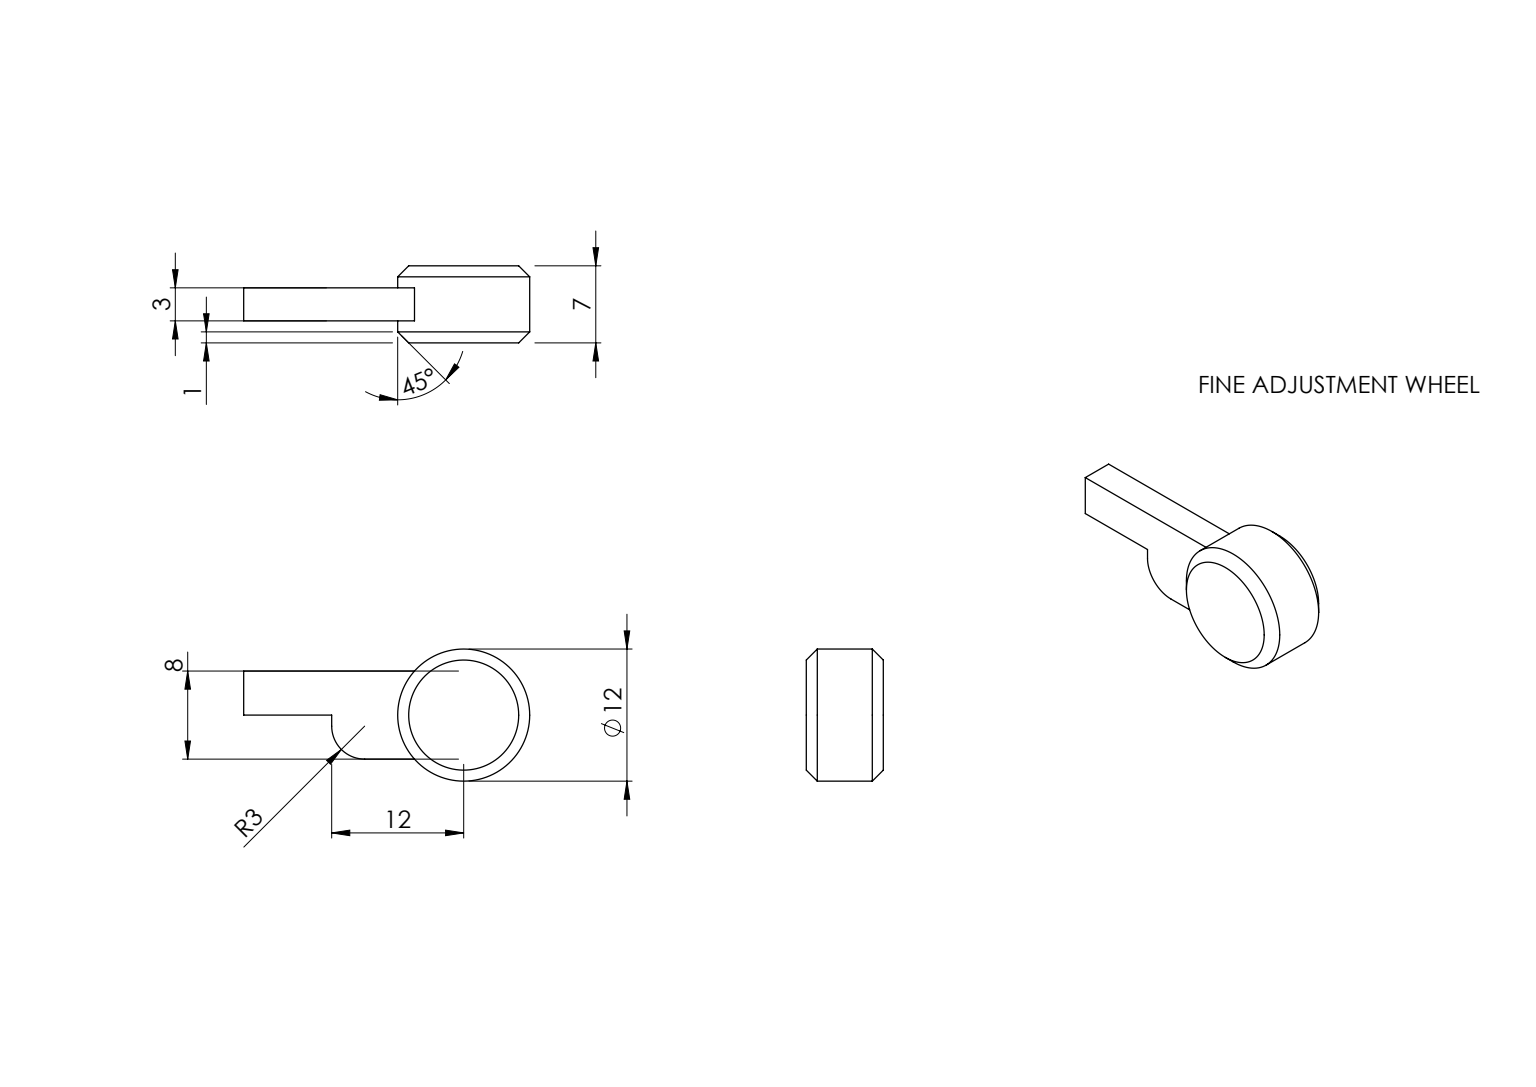
ISO-10303-21;
HEADER;
FILE_DESCRIPTION (('STEP AP214'),
    '1' );
FILE_NAME ('fine adjustment wheel.step',
    '2026-10-27T04:40:18',
    ( '' ),
    ( '' ),
    'SwSTEP 2.0',
    'SolidWorks 2026',
    '' );
FILE_SCHEMA (( 'AUTOMOTIVE_DESIGN' ));
ENDSEC;

DATA;
#10=ORIENTED_EDGE ( 'NONE', *, *, #8889, .F. ) ;
#13=ADVANCED_FACE ( 'NONE', ( #1458 ), #5708, .T. ) ;
#36=DIRECTION ( 'NONE',  ( 1.000000000000000000, 0.000000000000000000, 0.000000000000000000 ) ) ;
#47=DIRECTION ( 'NONE',  ( -0.000000000000000000, -0.000000000000000000, -1.000000000000000000 ) ) ;
#49=EDGE_LOOP ( 'NONE', ( #4259, #9067, #9089, #3500, #4349, #3630, #6139, #9782 ) ) ;
#70=CARTESIAN_POINT ( 'NONE',  ( -37.99999999999999289, -14.00000000000000888, -2.000000000000000000 ) ) ;
#86=ORIENTED_EDGE ( 'NONE', *, *, #4258, .T. ) ;
#91=EDGE_CURVE ( 'NONE', #7478, #353, #1465, .T. ) ;
#153=EDGE_CURVE ( 'NONE', #9355, #9315, #9914, .T. ) ;
#179=ADVANCED_BREP_SHAPE_REPRESENTATION ( '', ( #4912, #2307 ), #5679 ) ;
#216=ORIENTED_EDGE ( 'NONE', *, *, #8132, .T. ) ;
#224=VECTOR ( 'NONE', #3060, 999.9999999999998863 ) ;
#242=AXIS2_PLACEMENT_3D ( 'NONE', #968, #2330, #9109 ) ;
#274=LINE ( 'NONE', #989, #4138 ) ;
#291=CARTESIAN_POINT ( 'NONE',  ( -49.99999999999998579, -14.00000000000001243, 0.000000000000000000 ) ) ;
#300=ORIENTED_EDGE ( 'NONE', *, *, #8132, .F. ) ;
#327=AXIS2_PLACEMENT_3D ( 'NONE', #3024, #4508, #7911 ) ;
#339=EDGE_CURVE ( 'NONE', #1405, #2680, #6609, .T. ) ;
#353=VERTEX_POINT ( 'NONE', #8565 ) ;
#365=STYLED_ITEM ( 'NONE', ( #4697 ), #179 ) ;
#405=ORIENTED_EDGE ( 'NONE', *, *, #8852, .F. ) ;
#438=ORIENTED_EDGE ( 'NONE', *, *, #7786, .T. ) ;
#508=EDGE_CURVE ( 'NONE', #7478, #5442, #2848, .T. ) ;
#517=ORIENTED_EDGE ( 'NONE', *, *, #8212, .T. ) ;
#530=SHAPE_DEFINITION_REPRESENTATION ( #1480, #9271 ) ;
#531=DIRECTION ( 'NONE',  ( -1.000000000000000000, 0.000000000000000000, 0.000000000000000000 ) ) ;
#580=AXIS2_PLACEMENT_3D ( 'NONE', #1728, #9502, #4442 ) ;
#618=CARTESIAN_POINT ( 'NONE',  ( -37.99999999999999289, -14.00000000000000888, -0.9999999999999947820 ) ) ;
#626=CARTESIAN_POINT ( 'NONE',  ( -37.99999999999999289, -14.00000000000000888, -0.9999999999999947820 ) ) ;
#627=FACE_OUTER_BOUND ( 'NONE', #8133, .T. ) ;
#640=ADVANCED_FACE ( 'NONE', ( #10832 ), #2433, .T. ) ;
#668=CIRCLE ( 'NONE', #1009, 3.000000000000002665 ) ;
#712=EDGE_LOOP ( 'NONE', ( #5700, #5291 ) ) ;
#713=CARTESIAN_POINT ( 'NONE',  ( -57.99999999999998579, -10.00000000000000888, 0.000000000000000000 ) ) ;
#741=EDGE_CURVE ( 'NONE', #9355, #2941, #7719, .T. ) ;
#812=ORIENTED_EDGE ( 'NONE', *, *, #91, .F. ) ;
#866=CARTESIAN_POINT ( 'NONE',  ( -49.99999999999998579, -14.00000000000001243, 3.000000000000000000 ) ) ;
#903=DIRECTION ( 'NONE',  ( -1.000000000000000000, 0.000000000000000000, 0.000000000000000000 ) ) ;
#908=CARTESIAN_POINT ( 'NONE',  ( -43.00000000000000711, -14.00000000000000888, 5.000000000000000000 ) ) ;
#931=FACE_OUTER_BOUND ( 'NONE', #8908, .T. ) ;
#933=ORIENTED_EDGE ( 'NONE', *, *, #3473, .F. ) ;
#937=DIRECTION ( 'NONE',  ( -0.000000000000000000, -0.000000000000000000, -1.000000000000000000 ) ) ;
#968=CARTESIAN_POINT ( 'NONE',  ( -46.99999999999998579, -15.00000000000001066, 0.000000000000000000 ) ) ;
#989=CARTESIAN_POINT ( 'NONE',  ( -31.99999999999998579, -14.00000000000000888, -0.9999999999999947820 ) ) ;
#1001=APPLICATION_CONTEXT ( 'automotive_design' ) ;
#1009=AXIS2_PLACEMENT_3D ( 'NONE', #2485, #7596, #1705 ) ;
#1111=CARTESIAN_POINT ( 'NONE',  ( -46.99999999999998579, -18.00000000000001066, 0.000000000000000000 ) ) ;
#1122=CIRCLE ( 'NONE', #2538, 6.000000000000005329 ) ;
#1146=LINE ( 'NONE', #4527, #1576 ) ;
#1201=( NAMED_UNIT ( * ) SI_UNIT ( $, .STERADIAN. ) SOLID_ANGLE_UNIT ( ) );
#1208=DIRECTION ( 'NONE',  ( -0.000000000000000000, 0.000000000000000000, 1.000000000000000000 ) ) ;
#1210=DIRECTION ( 'NONE',  ( -0.000000000000000000, -0.000000000000000000, -1.000000000000000000 ) ) ;
#1256=MECHANICAL_DESIGN_GEOMETRIC_PRESENTATION_REPRESENTATION('',(#365),#3726);
#1265=SURFACE_SIDE_STYLE ('',( #8878 ) ) ;
#1327=SURFACE_STYLE_USAGE ( .BOTH. , #1265 ) ;
#1350=LINE ( 'NONE', #3214, #9205 ) ;
#1354=ORIENTED_EDGE ( 'NONE', *, *, #2995, .F. ) ;
#1391=CARTESIAN_POINT ( 'NONE',  ( -43.00000000000000711, -14.00000000000000888, 5.000000000000000000 ) ) ;
#1400=DIRECTION ( 'NONE',  ( 0.000000000000000000, 0.000000000000000000, 1.000000000000000000 ) ) ;
#1405=VERTEX_POINT ( 'NONE', #2148 ) ;
#1445=DIRECTION ( 'NONE',  ( 1.000000000000000000, 0.000000000000000000, 0.000000000000000000 ) ) ;
#1458=FACE_OUTER_BOUND ( 'NONE', #2511, .T. ) ;
#1462=( NAMED_UNIT ( * ) PLANE_ANGLE_UNIT ( ) SI_UNIT ( $, .RADIAN. ) );
#1465=CIRCLE ( 'NONE', #4462, 6.000000000000005329 ) ;
#1480=PRODUCT_DEFINITION_SHAPE ( 'NONE', 'NONE',  #3253 ) ;
#1506=DIRECTION ( 'NONE',  ( 0.000000000000000000, -1.000000000000000000, 0.000000000000000000 ) ) ;
#1550=EDGE_CURVE ( 'NONE', #3881, #2721, #10065, .T. ) ;
#1552=DIRECTION ( 'NONE',  ( 1.000000000000000000, 0.000000000000000000, -0.000000000000000000 ) ) ;
#1576=VECTOR ( 'NONE', #6088, 1000.000000000000000 ) ;
#1590=ORIENTED_EDGE ( 'NONE', *, *, #8473, .F. ) ;
#1597=LINE ( 'NONE', #10875, #4744 ) ;
#1613=DIRECTION ( 'NONE',  ( 0.000000000000000000, 0.000000000000000000, -1.000000000000000000 ) ) ;
#1629=CLOSED_SHELL ( 'NONE', ( #3641, #13, #7424, #7023, #3241, #9816, #9154, #8281, #8359, #2977, #2527, #640, #4769, #7997, #5715, #2128 ) ) ;
#1683=PLANE ( 'NONE',  #2131 ) ;
#1705=DIRECTION ( 'NONE',  ( 1.000000000000000000, 0.000000000000000000, 0.000000000000000000 ) ) ;
#1706=DIRECTION ( 'NONE',  ( 1.000000000000000000, 0.000000000000000000, 0.000000000000000000 ) ) ;
#1728=CARTESIAN_POINT ( 'NONE',  ( -37.99999999999999289, -14.00000000000000888, -2.000000000000000000 ) ) ;
#1738=DIRECTION ( 'NONE',  ( 0.000000000000000000, 0.000000000000000000, 1.000000000000000000 ) ) ;
#1745=FACE_OUTER_BOUND ( 'NONE', #9362, .T. ) ;
#1753=LINE ( 'NONE', #4344, #8240 ) ;
#1799=CARTESIAN_POINT ( 'NONE',  ( -46.99999999999998579, -15.00000000000001066, 3.000000000000000000 ) ) ;
#1808=CARTESIAN_POINT ( 'NONE',  ( -42.47213595499957961, -18.00000000000001066, 3.000000000000000000 ) ) ;
#1866=CARTESIAN_POINT ( 'NONE',  ( -49.99999999999998579, -18.00000000000001066, 3.000000000000000000 ) ) ;
#1873=APPLICATION_CONTEXT ( 'automotive_design' ) ;
#1881=FACE_OUTER_BOUND ( 'NONE', #4804, .T. ) ;
#1932=ORIENTED_EDGE ( 'NONE', *, *, #7786, .F. ) ;
#1992=DIRECTION ( 'NONE',  ( -0.000000000000000000, 0.000000000000000000, -1.000000000000000000 ) ) ;
#2011=LINE ( 'NONE', #3612, #5286 ) ;
#2028=AXIS2_PLACEMENT_3D ( 'NONE', #10381, #937, #2725 ) ;
#2094=DIRECTION ( 'NONE',  ( 0.000000000000000000, -0.000000000000000000, 1.000000000000000000 ) ) ;
#2101=CARTESIAN_POINT ( 'NONE',  ( 0.000000000000000000, 0.000000000000000000, 3.000000000000000000 ) ) ;
#2128=ADVANCED_FACE ( 'NONE', ( #1745 ), #2802, .T. ) ;
#2131=AXIS2_PLACEMENT_3D ( 'NONE', #7736, #5056, #2617 ) ;
#2148=CARTESIAN_POINT ( 'NONE',  ( -32.99999999999998579, -14.00000000000000888, -2.000000000000000000 ) ) ;
#2186=DIRECTION ( 'NONE',  ( 1.000000000000000000, -1.734723475976805517E-15, 0.000000000000000000 ) ) ;
#2199=FACE_OUTER_BOUND ( 'NONE', #4921, .T. ) ;
#2301=DIRECTION ( 'NONE',  ( 0.000000000000000000, 0.000000000000000000, -1.000000000000000000 ) ) ;
#2307=AXIS2_PLACEMENT_3D ( 'NONE', #5193, #3646, #1706 ) ;
#2314=CIRCLE ( 'NONE', #9227, 6.000000000000005329 ) ;
#2330=DIRECTION ( 'NONE',  ( 0.000000000000000000, -0.000000000000000000, -1.000000000000000000 ) ) ;
#2337=LINE ( 'NONE', #9118, #4782 ) ;
#2343=VECTOR ( 'NONE', #8296, 1000.000000000000000 ) ;
#2349=DIRECTION ( 'NONE',  ( 0.000000000000000000, 0.000000000000000000, -1.000000000000000000 ) ) ;
#2386=DIRECTION ( 'NONE',  ( -0.000000000000000000, -0.000000000000000000, 1.000000000000000000 ) ) ;
#2387=DIRECTION ( 'NONE',  ( -1.000000000000000000, 0.000000000000000000, 0.000000000000000000 ) ) ;
#2402=DIRECTION ( 'NONE',  ( 0.000000000000000000, 0.000000000000000000, 1.000000000000000000 ) ) ;
#2428=AXIS2_PLACEMENT_3D ( 'NONE', #6380, #8939, #3823 ) ;
#2433=PLANE ( 'NONE',  #7154 ) ;
#2436=EDGE_CURVE ( 'NONE', #4203, #4184, #3595, .T. ) ;
#2442=( LENGTH_UNIT ( ) NAMED_UNIT ( * ) SI_UNIT ( .MILLI., .METRE. ) );
#2454=CARTESIAN_POINT ( 'NONE',  ( -44.00000000000000000, -14.00000000000000888, -0.9999999999999947820 ) ) ;
#2457=EDGE_CURVE ( 'NONE', #5442, #2721, #1122, .T. ) ;
#2458=CONICAL_SURFACE ( 'NONE', #10080, 5.000000000000018652, 0.7853981633974430610 ) ;
#2485=CARTESIAN_POINT ( 'NONE',  ( -46.99999999999998579, -15.00000000000001066, 3.000000000000000000 ) ) ;
#2507=DIRECTION ( 'NONE',  ( -0.000000000000000000, -0.000000000000000000, -1.000000000000000000 ) ) ;
#2511=EDGE_LOOP ( 'NONE', ( #1590, #7595, #1354, #8774 ) ) ;
#2527=ADVANCED_FACE ( 'NONE', ( #9231 ), #2606, .T. ) ;
#2538=AXIS2_PLACEMENT_3D ( 'NONE', #5888, #3381, #8289 ) ;
#2606=CYLINDRICAL_SURFACE ( 'NONE', #2028, 6.000000000000005329 ) ;
#2617=DIRECTION ( 'NONE',  ( 0.000000000000000000, -0.000000000000000000, -1.000000000000000000 ) ) ;
#2647=EDGE_CURVE ( 'NONE', #1405, #9106, #274, .T. ) ;
#2657=ORIENTED_EDGE ( 'NONE', *, *, #6128, .F. ) ;
#2673=DIRECTION ( 'NONE',  ( 0.000000000000000000, -0.000000000000000000, 1.000000000000000000 ) ) ;
#2680=VERTEX_POINT ( 'NONE', #5150 ) ;
#2690=DIRECTION ( 'NONE',  ( -0.000000000000000000, 0.000000000000000000, -1.000000000000000000 ) ) ;
#2691=ORIENTED_EDGE ( 'NONE', *, *, #2647, .T. ) ;
#2712=ORIENTED_EDGE ( 'NONE', *, *, #339, .F. ) ;
#2721=VERTEX_POINT ( 'NONE', #9785 ) ;
#2722=AXIS2_PLACEMENT_3D ( 'NONE', #618, #6864, #3357 ) ;
#2725=DIRECTION ( 'NONE',  ( -1.000000000000000000, 0.000000000000000000, 0.000000000000000000 ) ) ;
#2734=VERTEX_POINT ( 'NONE', #6508 ) ;
#2768=CARTESIAN_POINT ( 'NONE',  ( -57.99999999999998579, -10.00000000000000888, 3.000000000000000000 ) ) ;
#2793=EDGE_CURVE ( 'NONE', #4184, #353, #7173, .T. ) ;
#2795=ORIENTED_EDGE ( 'NONE', *, *, #8073, .T. ) ;
#2802=CYLINDRICAL_SURFACE ( 'NONE', #5740, 3.000000000000002665 ) ;
#2819=CARTESIAN_POINT ( 'NONE',  ( -57.99999999999998579, -10.00000000000000888, 0.000000000000000000 ) ) ;
#2834=ORIENTED_EDGE ( 'NONE', *, *, #7357, .T. ) ;
#2848=LINE ( 'NONE', #10615, #9097 ) ;
#2850=DIRECTION ( 'NONE',  ( 0.000000000000000000, -0.000000000000000000, -1.000000000000000000 ) ) ;
#2880=CARTESIAN_POINT ( 'NONE',  ( -49.99999999999998579, -14.00000000000001243, 3.000000000000000000 ) ) ;
#2902=EDGE_CURVE ( 'NONE', #3086, #4883, #1753, .T. ) ;
#2916=LINE ( 'NONE', #6304, #5810 ) ;
#2941=VERTEX_POINT ( 'NONE', #1808 ) ;
#2959=DIRECTION ( 'NONE',  ( 0.000000000000000000, -1.000000000000000000, 0.000000000000000000 ) ) ;
#2977=ADVANCED_FACE ( 'NONE', ( #6925 ), #3524, .F. ) ;
#2995=EDGE_CURVE ( 'NONE', #9106, #8034, #6093, .T. ) ;
#3004=MECHANICAL_DESIGN_GEOMETRIC_PRESENTATION_REPRESENTATION('',(#6552),#5273);
#3024=CARTESIAN_POINT ( 'NONE',  ( -37.99999999999999289, -14.00000000000000888, -0.9999999999999947820 ) ) ;
#3034=ORIENTED_EDGE ( 'NONE', *, *, #2793, .F. ) ;
#3060=DIRECTION ( 'NONE',  ( -0.7071067811865439090, 0.000000000000000000, -0.7071067811865512365 ) ) ;
#3069=ORIENTED_EDGE ( 'NONE', *, *, #8889, .T. ) ;
#3077=ORIENTED_EDGE ( 'NONE', *, *, #2902, .T. ) ;
#3078=CARTESIAN_POINT ( 'NONE',  ( -31.99999999999997868, -14.00000000000000888, -0.9999999999999947820 ) ) ;
#3086=VERTEX_POINT ( 'NONE', #5179 ) ;
#3094=EDGE_CURVE ( 'NONE', #9315, #7434, #8946, .T. ) ;
#3096=( NAMED_UNIT ( * ) PLANE_ANGLE_UNIT ( ) SI_UNIT ( $, .RADIAN. ) );
#3135=DIRECTION ( 'NONE',  ( 1.000000000000000000, 0.000000000000000000, 0.000000000000000000 ) ) ;
#3175=DIRECTION ( 'NONE',  ( 1.000000000000000000, 0.000000000000000000, 0.000000000000000000 ) ) ;
#3214=CARTESIAN_POINT ( 'NONE',  ( -57.99999999999998579, -10.00000000000000888, 3.000000000000000000 ) ) ;
#3241=ADVANCED_FACE ( 'NONE', ( #9702 ), #6981, .F. ) ;
#3253=PRODUCT_DEFINITION ( 'UNKNOWN', '', #7291, #4620 ) ;
#3271=UNCERTAINTY_MEASURE_WITH_UNIT (LENGTH_MEASURE( 1.000000000000000082E-05 ), #2442, 'distance_accuracy_value', 'NONE');
#3305=EDGE_CURVE ( 'NONE', #5709, #3086, #6491, .T. ) ;
#3337=ORIENTED_EDGE ( 'NONE', *, *, #3473, .T. ) ;
#3357=DIRECTION ( 'NONE',  ( 1.000000000000000000, 0.000000000000000000, 0.000000000000000000 ) ) ;
#3381=DIRECTION ( 'NONE',  ( 0.000000000000000000, -0.000000000000000000, -1.000000000000000000 ) ) ;
#3386=LINE ( 'NONE', #3496, #3889 ) ;
#3430=DIRECTION ( 'NONE',  ( 1.000000000000000000, 0.000000000000000000, 0.000000000000000000 ) ) ;
#3439=CARTESIAN_POINT ( 'NONE',  ( -57.99999999999998579, -14.00000000000001243, 3.000000000000000000 ) ) ;
#3473=EDGE_CURVE ( 'NONE', #2734, #7921, #9567, .T. ) ;
#3496=CARTESIAN_POINT ( 'NONE',  ( -44.00000000000000000, -14.00000000000000888, 5.000000000000000000 ) ) ;
#3497=VECTOR ( 'NONE', #7882, 1000.000000000000000 ) ;
#3500=ORIENTED_EDGE ( 'NONE', *, *, #8212, .F. ) ;
#3524=PLANE ( 'NONE',  #8061 ) ;
#3534=COLOUR_RGB ( '',0.8941176470588234615, 0.8941176470588234615, 0.8941176470588234615 ) ;
#3583=AXIS2_PLACEMENT_3D ( 'NONE', #1866, #4468, #2094 ) ;
#3595=CIRCLE ( 'NONE', #5912, 5.000000000000018652 ) ;
#3612=CARTESIAN_POINT ( 'NONE',  ( -49.99999999999998579, -10.00000000000000888, 0.000000000000000000 ) ) ;
#3630=ORIENTED_EDGE ( 'NONE', *, *, #7165, .T. ) ;
#3641=ADVANCED_FACE ( 'NONE', ( #627 ), #8743, .T. ) ;
#3646=DIRECTION ( 'NONE',  ( 0.000000000000000000, 0.000000000000000000, 1.000000000000000000 ) ) ;
#3689=CARTESIAN_POINT ( 'NONE',  ( -32.99999999999997158, -14.00000000000000888, 5.000000000000000000 ) ) ;
#3726=( GEOMETRIC_REPRESENTATION_CONTEXT ( 3 ) GLOBAL_UNCERTAINTY_ASSIGNED_CONTEXT ( ( #7376 ) ) GLOBAL_UNIT_ASSIGNED_CONTEXT ( ( #8986, #3096, #4859 ) ) REPRESENTATION_CONTEXT ( 'NONE', 'WORKASPACE' ) );
#3774=VECTOR ( 'NONE', #3430, 1000.000000000000000 ) ;
#3809=EDGE_LOOP ( 'NONE', ( #3826, #2795, #9159, #7912 ) ) ;
#3822=VERTEX_POINT ( 'NONE', #7558 ) ;
#3823=DIRECTION ( 'NONE',  ( 1.000000000000000000, 0.000000000000000000, 0.000000000000000000 ) ) ;
#3826=ORIENTED_EDGE ( 'NONE', *, *, #6064, .T. ) ;
#3868=CIRCLE ( 'NONE', #9899, 5.000000000000018652 ) ;
#3878=DIRECTION ( 'NONE',  ( 0.000000000000000000, 0.000000000000000000, 1.000000000000000000 ) ) ;
#3881=VERTEX_POINT ( 'NONE', #5991 ) ;
#3889=VECTOR ( 'NONE', #2507, 1000.000000000000000 ) ;
#3906=AXIS2_PLACEMENT_3D ( 'NONE', #6884, #47, #10933 ) ;
#3915=CONICAL_SURFACE ( 'NONE', #5308, 6.000000000000005329, 0.7853981633974479459 ) ;
#3938=DIRECTION ( 'NONE',  ( 0.000000000000000000, -1.000000000000000000, 0.000000000000000000 ) ) ;
#3949=AXIS2_PLACEMENT_3D ( 'NONE', #10889, #1613, #2387 ) ;
#4033=CIRCLE ( 'NONE', #4565, 5.000000000000004441 ) ;
#4087=EDGE_CURVE ( 'NONE', #4203, #7478, #9887, .T. ) ;
#4127=VECTOR ( 'NONE', #10514, 1000.000000000000000 ) ;
#4138=VECTOR ( 'NONE', #7055, 1000.000000000000000 ) ;
#4147=ORIENTED_EDGE ( 'NONE', *, *, #8394, .F. ) ;
#4156=ORIENTED_EDGE ( 'NONE', *, *, #2436, .T. ) ;
#4169=DIRECTION ( 'NONE',  ( -0.7071067811865472397, 8.659560562354929160E-17, 0.7071067811865479058 ) ) ;
#4184=VERTEX_POINT ( 'NONE', #3689 ) ;
#4186=DIRECTION ( 'NONE',  ( 1.000000000000000000, 0.000000000000000000, -0.000000000000000000 ) ) ;
#4203=VERTEX_POINT ( 'NONE', #908 ) ;
#4209=CARTESIAN_POINT ( 'NONE',  ( -37.99999999999999289, -14.00000000000000888, 5.000000000000000000 ) ) ;
#4258=EDGE_CURVE ( 'NONE', #5709, #8064, #6196, .T. ) ;
#4259=ORIENTED_EDGE ( 'NONE', *, *, #10324, .F. ) ;
#4302=DIRECTION ( 'NONE',  ( -0.000000000000000000, -0.000000000000000000, 1.000000000000000000 ) ) ;
#4344=CARTESIAN_POINT ( 'NONE',  ( -57.99999999999998579, -14.00000000000001243, 0.000000000000000000 ) ) ;
#4349=ORIENTED_EDGE ( 'NONE', *, *, #9274, .T. ) ;
#4351=CARTESIAN_POINT ( 'NONE',  ( -49.99999999999998579, -15.00000000000001066, 3.000000000000000000 ) ) ;
#4442=DIRECTION ( 'NONE',  ( 1.000000000000000000, 0.000000000000000000, 0.000000000000000000 ) ) ;
#4444=DIRECTION ( 'NONE',  ( 0.000000000000000000, -0.000000000000000000, -1.000000000000000000 ) ) ;
#4462=AXIS2_PLACEMENT_3D ( 'NONE', #8254, #2349, #3135 ) ;
#4468=DIRECTION ( 'NONE',  ( 0.000000000000000000, 1.000000000000000000, 0.000000000000000000 ) ) ;
#4488=EDGE_LOOP ( 'NONE', ( #4156, #7221 ) ) ;
#4505=CARTESIAN_POINT ( 'NONE',  ( -57.99999999999998579, -10.00000000000000888, 3.000000000000000000 ) ) ;
#4508=DIRECTION ( 'NONE',  ( -0.000000000000000000, -0.000000000000000000, 1.000000000000000000 ) ) ;
#4527=CARTESIAN_POINT ( 'NONE',  ( -31.99999999999998579, -14.00000000000000888, 5.000000000000000000 ) ) ;
#4556=EDGE_LOOP ( 'NONE', ( #3077, #9544, #5564, #9901 ) ) ;
#4563=DIRECTION ( 'NONE',  ( 0.000000000000000000, 0.000000000000000000, -1.000000000000000000 ) ) ;
#4565=AXIS2_PLACEMENT_3D ( 'NONE', #8826, #1210, #4591 ) ;
#4588=DIRECTION ( 'NONE',  ( 1.000000000000000000, 0.000000000000000000, 0.000000000000000000 ) ) ;
#4591=DIRECTION ( 'NONE',  ( 1.000000000000000000, 0.000000000000000000, 0.000000000000000000 ) ) ;
#4617=DIRECTION ( 'NONE',  ( -0.000000000000000000, -0.000000000000000000, -1.000000000000000000 ) ) ;
#4620=PRODUCT_DEFINITION_CONTEXT ( 'detailed design', #1873, 'design' ) ;
#4697=PRESENTATION_STYLE_ASSIGNMENT (( #1327 ) ) ;
#4729=ORIENTED_EDGE ( 'NONE', *, *, #1550, .T. ) ;
#4744=VECTOR ( 'NONE', #10038, 1000.000000000000000 ) ;
#4748=CARTESIAN_POINT ( 'NONE',  ( -57.99999999999998579, -14.00000000000001243, 3.000000000000000000 ) ) ;
#4749=FILL_AREA_STYLE_COLOUR ( '', #3534 ) ;
#4769=ADVANCED_FACE ( 'NONE', ( #6123 ), #9345, .F. ) ;
#4782=VECTOR ( 'NONE', #1506, 1000.000000000000000 ) ;
#4804=EDGE_LOOP ( 'NONE', ( #438, #8620, #6062, #3337 ) ) ;
#4808=PLANE ( 'NONE',  #2428 ) ;
#4859=( NAMED_UNIT ( * ) SI_UNIT ( $, .STERADIAN. ) SOLID_ANGLE_UNIT ( ) );
#4883=VERTEX_POINT ( 'NONE', #291 ) ;
#4887=( NAMED_UNIT ( * ) SI_UNIT ( $, .STERADIAN. ) SOLID_ANGLE_UNIT ( ) );
#4892=EDGE_CURVE ( 'NONE', #8034, #9106, #8658, .T. ) ;
#4912=MANIFOLD_SOLID_BREP ( 'Fillet1', #1629 ) ;
#4921=EDGE_LOOP ( 'NONE', ( #3034, #7353, #9276, #405 ) ) ;
#4980=AXIS2_PLACEMENT_3D ( 'NONE', #70, #1738, #5112 ) ;
#4994=DIRECTION ( 'NONE',  ( 0.000000000000000000, 1.000000000000000000, 0.000000000000000000 ) ) ;
#5056=DIRECTION ( 'NONE',  ( 0.000000000000000000, -1.000000000000000000, 0.000000000000000000 ) ) ;
#5112=DIRECTION ( 'NONE',  ( 1.000000000000000000, 0.000000000000000000, -0.000000000000000000 ) ) ;
#5150=CARTESIAN_POINT ( 'NONE',  ( -43.00000000000000000, -14.00000000000000888, -2.000000000000000000 ) ) ;
#5176=CARTESIAN_POINT ( 'NONE',  ( -57.99999999999998579, -14.00000000000001243, 3.000000000000000000 ) ) ;
#5177=ORIENTED_EDGE ( 'NONE', *, *, #10324, .T. ) ;
#5178=VECTOR ( 'NONE', #2402, 1000.000000000000000 ) ;
#5179=CARTESIAN_POINT ( 'NONE',  ( -57.99999999999998579, -14.00000000000001243, 0.000000000000000000 ) ) ;
#5190=LINE ( 'NONE', #4351, #6219 ) ;
#5193=CARTESIAN_POINT ( 'NONE',  ( 0.000000000000000000, 0.000000000000000000, 0.000000000000000000 ) ) ;
#5201=ORIENTED_EDGE ( 'NONE', *, *, #7114, .T. ) ;
#5244=PLANE ( 'NONE',  #8470 ) ;
#5273=( GEOMETRIC_REPRESENTATION_CONTEXT ( 3 ) GLOBAL_UNCERTAINTY_ASSIGNED_CONTEXT ( ( #3271 ) ) GLOBAL_UNIT_ASSIGNED_CONTEXT ( ( #2442, #1462, #4887 ) ) REPRESENTATION_CONTEXT ( 'NONE', 'WORKASPACE' ) );
#5284=ORIENTED_EDGE ( 'NONE', *, *, #2793, .T. ) ;
#5286=VECTOR ( 'NONE', #2959, 1000.000000000000000 ) ;
#5291=ORIENTED_EDGE ( 'NONE', *, *, #8473, .T. ) ;
#5308=AXIS2_PLACEMENT_3D ( 'NONE', #5814, #4302, #36 ) ;
#5374=VECTOR ( 'NONE', #9002, 999.9999999999998863 ) ;
#5442=VERTEX_POINT ( 'NONE', #10043 ) ;
#5545=ORIENTED_EDGE ( 'NONE', *, *, #4892, .F. ) ;
#5564=ORIENTED_EDGE ( 'NONE', *, *, #4258, .F. ) ;
#5573=ORIENTED_EDGE ( 'NONE', *, *, #741, .T. ) ;
#5577=CARTESIAN_POINT ( 'NONE',  ( -37.99999999999999289, -14.00000000000000888, 5.000000000000000000 ) ) ;
#5642=DIRECTION ( 'NONE',  ( -0.000000000000000000, -0.000000000000000000, -1.000000000000000000 ) ) ;
#5658=ORIENTED_EDGE ( 'NONE', *, *, #8113, .T. ) ;
#5666=DIRECTION ( 'NONE',  ( -1.000000000000000000, -0.000000000000000000, -0.000000000000000000 ) ) ;
#5673=CIRCLE ( 'NONE', #8339, 6.000000000000005329 ) ;
#5679=( GEOMETRIC_REPRESENTATION_CONTEXT ( 3 ) GLOBAL_UNCERTAINTY_ASSIGNED_CONTEXT ( ( #6600 ) ) GLOBAL_UNIT_ASSIGNED_CONTEXT ( ( #10706, #10646, #1201 ) ) REPRESENTATION_CONTEXT ( 'NONE', 'WORKASPACE' ) );
#5689=LINE ( 'NONE', #2454, #9044 ) ;
#5694=EDGE_LOOP ( 'NONE', ( #10, #9413, #7170, #5973, #1932, #8095, #6662, #7528 ) ) ;
#5700=ORIENTED_EDGE ( 'NONE', *, *, #339, .T. ) ;
#5708=CONICAL_SURFACE ( 'NONE', #6255, 6.000000000000005329, 0.7853981633974479459 ) ;
#5709=VERTEX_POINT ( 'NONE', #7305 ) ;
#5715=ADVANCED_FACE ( 'NONE', ( #2199 ), #2458, .T. ) ;
#5740=AXIS2_PLACEMENT_3D ( 'NONE', #1799, #2690, #903 ) ;
#5761=ORIENTED_EDGE ( 'NONE', *, *, #2457, .F. ) ;
#5810=VECTOR ( 'NONE', #9686, 1000.000000000000000 ) ;
#5814=CARTESIAN_POINT ( 'NONE',  ( -37.99999999999999289, -14.00000000000000888, -0.9999999999999947820 ) ) ;
#5846=CARTESIAN_POINT ( 'NONE',  ( -42.47213595499957961, -10.00000000000000888, 5.000000000000000000 ) ) ;
#5870=CARTESIAN_POINT ( 'NONE',  ( -44.00000000000000711, -14.00000000000000888, -0.9999999999999947820 ) ) ;
#5884=ORIENTED_EDGE ( 'NONE', *, *, #153, .F. ) ;
#5886=EDGE_CURVE ( 'NONE', #6102, #8034, #3386, .T. ) ;
#5888=CARTESIAN_POINT ( 'NONE',  ( -37.99999999999999289, -14.00000000000000888, 3.000000000000000000 ) ) ;
#5901=FACE_OUTER_BOUND ( 'NONE', #6795, .T. ) ;
#5912=AXIS2_PLACEMENT_3D ( 'NONE', #4209, #10158, #3175 ) ;
#5937=CARTESIAN_POINT ( 'NONE',  ( -49.99999999999998579, -15.00000000000001066, 0.000000000000000000 ) ) ;
#5973=ORIENTED_EDGE ( 'NONE', *, *, #2902, .F. ) ;
#5987=AXIS2_PLACEMENT_3D ( 'NONE', #8089, #4563, #8917 ) ;
#5991=CARTESIAN_POINT ( 'NONE',  ( -42.47213595499957961, -10.00000000000000888, 0.000000000000000000 ) ) ;
#6062=ORIENTED_EDGE ( 'NONE', *, *, #7357, .F. ) ;
#6064=EDGE_CURVE ( 'NONE', #4883, #7434, #2011, .T. ) ;
#6088=DIRECTION ( 'NONE',  ( -0.000000000000000000, -0.000000000000000000, -1.000000000000000000 ) ) ;
#6093=CIRCLE ( 'NONE', #2722, 6.000000000000005329 ) ;
#6102=VERTEX_POINT ( 'NONE', #9005 ) ;
#6123=FACE_OUTER_BOUND ( 'NONE', #712, .T. ) ;
#6128=EDGE_CURVE ( 'NONE', #2721, #2734, #1350, .T. ) ;
#6139=ORIENTED_EDGE ( 'NONE', *, *, #5886, .T. ) ;
#6196=LINE ( 'NONE', #5176, #8387 ) ;
#6219=VECTOR ( 'NONE', #9210, 1000.000000000000000 ) ;
#6255=AXIS2_PLACEMENT_3D ( 'NONE', #626, #2386, #10781 ) ;
#6268=DIRECTION ( 'NONE',  ( -1.000000000000000000, -0.000000000000000000, -0.000000000000000000 ) ) ;
#6273=DIRECTION ( 'NONE',  ( 1.000000000000000000, 0.000000000000000000, -0.000000000000000000 ) ) ;
#6304=CARTESIAN_POINT ( 'NONE',  ( -49.99999999999998579, -18.00000000000001066, 0.000000000000000000 ) ) ;
#6380=CARTESIAN_POINT ( 'NONE',  ( 0.000000000000000000, 0.000000000000000000, 0.000000000000000000 ) ) ;
#6452=VERTEX_POINT ( 'NONE', #7542 ) ;
#6491=LINE ( 'NONE', #4748, #8380 ) ;
#6508=CARTESIAN_POINT ( 'NONE',  ( -57.99999999999998579, -10.00000000000000888, 3.000000000000000000 ) ) ;
#6514=CARTESIAN_POINT ( 'NONE',  ( -37.99999999999999289, -14.00000000000000888, 5.000000000000000000 ) ) ;
#6549=EDGE_CURVE ( 'NONE', #3881, #7921, #9593, .T. ) ;
#6552=STYLED_ITEM('',(#11006),#4912);
#6562=ORIENTED_EDGE ( 'NONE', *, *, #1550, .F. ) ;
#6599=SHAPE_REPRESENTATION_RELATIONSHIP ( 'NONE' , 'NONE' ,  #9271, #179 ) ;
#6600=UNCERTAINTY_MEASURE_WITH_UNIT (LENGTH_MEASURE( 1.000000000000000082E-05 ), #10706, 'distance_accuracy_value', 'NONE');
#6609=CIRCLE ( 'NONE', #580, 5.000000000000004441 ) ;
#6662=ORIENTED_EDGE ( 'NONE', *, *, #7114, .F. ) ;
#6688=EDGE_CURVE ( 'NONE', #2680, #8034, #5689, .T. ) ;
#6716=AXIS2_PLACEMENT_3D ( 'NONE', #2768, #6273, #1992 ) ;
#6795=EDGE_LOOP ( 'NONE', ( #6562, #7112, #933, #2657 ) ) ;
#6815=EDGE_LOOP ( 'NONE', ( #5658, #216, #5573, #517, #8607, #10223, #2834, #86 ) ) ;
#6864=DIRECTION ( 'NONE',  ( -0.000000000000000000, -0.000000000000000000, 1.000000000000000000 ) ) ;
#6884=CARTESIAN_POINT ( 'NONE',  ( -37.99999999999999289, -14.00000000000000888, 5.000000000000000000 ) ) ;
#6925=FACE_OUTER_BOUND ( 'NONE', #3809, .T. ) ;
#6981=PLANE ( 'NONE',  #3583 ) ;
#7023=ADVANCED_FACE ( 'NONE', ( #5901 ), #1683, .F. ) ;
#7040=DIRECTION ( 'NONE',  ( 0.000000000000000000, -0.000000000000000000, -1.000000000000000000 ) ) ;
#7055=DIRECTION ( 'NONE',  ( 0.7071067811865472397, 0.000000000000000000, 0.7071067811865479058 ) ) ;
#7057=CARTESIAN_POINT ( 'NONE',  ( -42.47213595499957961, -18.00000000000001066, 5.000000000000000000 ) ) ;
#7102=LINE ( 'NONE', #2880, #3497 ) ;
#7108=PLANE ( 'NONE',  #6716 ) ;
#7112=ORIENTED_EDGE ( 'NONE', *, *, #6549, .T. ) ;
#7114=EDGE_CURVE ( 'NONE', #6102, #3881, #5673, .T. ) ;
#7154=AXIS2_PLACEMENT_3D ( 'NONE', #6514, #1400, #1552 ) ;
#7165=EDGE_CURVE ( 'NONE', #6452, #6102, #2314, .T. ) ;
#7170=ORIENTED_EDGE ( 'NONE', *, *, #6064, .F. ) ;
#7173=LINE ( 'NONE', #10668, #5374 ) ;
#7175=LINE ( 'NONE', #7057, #7768 ) ;
#7221=ORIENTED_EDGE ( 'NONE', *, *, #8394, .T. ) ;
#7269=DIRECTION ( 'NONE',  ( 1.000000000000000000, 0.000000000000000000, 0.000000000000000000 ) ) ;
#7291=PRODUCT_DEFINITION_FORMATION_WITH_SPECIFIED_SOURCE ( 'ANY', '', #7422, .NOT_KNOWN. ) ;
#7297=ORIENTED_EDGE ( 'NONE', *, *, #5886, .F. ) ;
#7305=CARTESIAN_POINT ( 'NONE',  ( -57.99999999999998579, -14.00000000000001243, 3.000000000000000000 ) ) ;
#7353=ORIENTED_EDGE ( 'NONE', *, *, #2436, .F. ) ;
#7357=EDGE_CURVE ( 'NONE', #2734, #5709, #2337, .T. ) ;
#7376=UNCERTAINTY_MEASURE_WITH_UNIT (LENGTH_MEASURE( 1.000000000000000082E-05 ), #8986, 'distance_accuracy_value', 'NONE');
#7378=FACE_OUTER_BOUND ( 'NONE', #5694, .T. ) ;
#7386=LINE ( 'NONE', #8998, #8168 ) ;
#7422=PRODUCT ( 'fine adjustment wheel', 'fine adjustment wheel', '', ( #8973 ) ) ;
#7424=ADVANCED_FACE ( 'NONE', ( #931 ), #9378, .T. ) ;
#7434=VERTEX_POINT ( 'NONE', #5937 ) ;
#7470=ORIENTED_EDGE ( 'NONE', *, *, #6688, .F. ) ;
#7478=VERTEX_POINT ( 'NONE', #8439 ) ;
#7506=ORIENTED_EDGE ( 'NONE', *, *, #741, .F. ) ;
#7528=ORIENTED_EDGE ( 'NONE', *, *, #7165, .F. ) ;
#7542=CARTESIAN_POINT ( 'NONE',  ( -42.47213595499957961, -18.00000000000001066, 0.000000000000000000 ) ) ;
#7543=ORIENTED_EDGE ( 'NONE', *, *, #9274, .F. ) ;
#7558=CARTESIAN_POINT ( 'NONE',  ( -49.99999999999998579, -15.00000000000001066, 3.000000000000000000 ) ) ;
#7585=AXIS2_PLACEMENT_3D ( 'NONE', #7821, #7040, #7936 ) ;
#7588=DIRECTION ( 'NONE',  ( -0.000000000000000000, 0.000000000000000000, -1.000000000000000000 ) ) ;
#7595=ORIENTED_EDGE ( 'NONE', *, *, #6688, .T. ) ;
#7596=DIRECTION ( 'NONE',  ( -0.000000000000000000, 0.000000000000000000, 1.000000000000000000 ) ) ;
#7719=LINE ( 'NONE', #10255, #3774 ) ;
#7736=CARTESIAN_POINT ( 'NONE',  ( -57.99999999999998579, -10.00000000000000888, 3.000000000000000000 ) ) ;
#7754=DIRECTION ( 'NONE',  ( 1.000000000000000000, 0.000000000000000000, 0.000000000000000000 ) ) ;
#7768=VECTOR ( 'NONE', #9554, 1000.000000000000000 ) ;
#7786=EDGE_CURVE ( 'NONE', #7921, #3086, #7386, .T. ) ;
#7821=CARTESIAN_POINT ( 'NONE',  ( -37.99999999999999289, -14.00000000000000888, 3.000000000000000000 ) ) ;
#7828=ORIENTED_EDGE ( 'NONE', *, *, #4087, .F. ) ;
#7837=CARTESIAN_POINT ( 'NONE',  ( -46.99999999999998579, -18.00000000000001066, 3.000000000000000000 ) ) ;
#7882=DIRECTION ( 'NONE',  ( -0.000000000000000000, -0.000000000000000000, -1.000000000000000000 ) ) ;
#7905=DIRECTION ( 'NONE',  ( 1.000000000000000000, 0.000000000000000000, 0.000000000000000000 ) ) ;
#7911=DIRECTION ( 'NONE',  ( 1.000000000000000000, 0.000000000000000000, 0.000000000000000000 ) ) ;
#7912=ORIENTED_EDGE ( 'NONE', *, *, #8187, .T. ) ;
#7921=VERTEX_POINT ( 'NONE', #713 ) ;
#7936=DIRECTION ( 'NONE',  ( 1.000000000000000000, 0.000000000000000000, 0.000000000000000000 ) ) ;
#7964=ORIENTED_EDGE ( 'NONE', *, *, #91, .T. ) ;
#7997=ADVANCED_FACE ( 'NONE', ( #8482 ), #3915, .T. ) ;
#8034=VERTEX_POINT ( 'NONE', #5870 ) ;
#8061=AXIS2_PLACEMENT_3D ( 'NONE', #10132, #4186, #7588 ) ;
#8064=VERTEX_POINT ( 'NONE', #866 ) ;
#8073=EDGE_CURVE ( 'NONE', #7434, #3822, #5190, .T. ) ;
#8089=CARTESIAN_POINT ( 'NONE',  ( -37.99999999999999289, -14.00000000000000888, 3.999999999999999112 ) ) ;
#8095=ORIENTED_EDGE ( 'NONE', *, *, #6549, .F. ) ;
#8108=CARTESIAN_POINT ( 'NONE',  ( -37.99999999999999289, -14.00000000000000888, 5.000000000000000000 ) ) ;
#8113=EDGE_CURVE ( 'NONE', #8064, #3822, #1597, .T. ) ;
#8132=EDGE_CURVE ( 'NONE', #3822, #9355, #668, .T. ) ;
#8133=EDGE_LOOP ( 'NONE', ( #4147, #5284, #812, #7828 ) ) ;
#8168=VECTOR ( 'NONE', #3938, 1000.000000000000000 ) ;
#8187=EDGE_CURVE ( 'NONE', #8064, #4883, #7102, .T. ) ;
#8212=EDGE_CURVE ( 'NONE', #2941, #5442, #10060, .T. ) ;
#8240=VECTOR ( 'NONE', #1445, 1000.000000000000000 ) ;
#8254=CARTESIAN_POINT ( 'NONE',  ( -37.99999999999999289, -14.00000000000000888, 3.999999999999999112 ) ) ;
#8281=ADVANCED_FACE ( 'NONE', ( #10419 ), #5244, .T. ) ;
#8289=DIRECTION ( 'NONE',  ( 1.000000000000000000, -1.734723475976805517E-15, 0.000000000000000000 ) ) ;
#8296=DIRECTION ( 'NONE',  ( -0.000000000000000000, 0.000000000000000000, -1.000000000000000000 ) ) ;
#8339=AXIS2_PLACEMENT_3D ( 'NONE', #9794, #2850, #2186 ) ;
#8359=ADVANCED_FACE ( 'NONE', ( #7378 ), #4808, .F. ) ;
#8380=VECTOR ( 'NONE', #5642, 1000.000000000000000 ) ;
#8387=VECTOR ( 'NONE', #7754, 1000.000000000000000 ) ;
#8394=EDGE_CURVE ( 'NONE', #4184, #4203, #3868, .T. ) ;
#8398=FACE_OUTER_BOUND ( 'NONE', #4556, .T. ) ;
#8439=CARTESIAN_POINT ( 'NONE',  ( -44.00000000000000711, -14.00000000000000888, 3.999999999999999112 ) ) ;
#8470=AXIS2_PLACEMENT_3D ( 'NONE', #2101, #1208, #4588 ) ;
#8473=EDGE_CURVE ( 'NONE', #2680, #1405, #4033, .T. ) ;
#8482=FACE_OUTER_BOUND ( 'NONE', #9603, .T. ) ;
#8484=ORIENTED_EDGE ( 'NONE', *, *, #3094, .F. ) ;
#8565=CARTESIAN_POINT ( 'NONE',  ( -31.99999999999997868, -14.00000000000000888, 3.999999999999999112 ) ) ;
#8607=ORIENTED_EDGE ( 'NONE', *, *, #2457, .T. ) ;
#8620=ORIENTED_EDGE ( 'NONE', *, *, #3305, .F. ) ;
#8658=CIRCLE ( 'NONE', #327, 6.000000000000005329 ) ;
#8743=CONICAL_SURFACE ( 'NONE', #3949, 5.000000000000018652, 0.7853981633974430610 ) ;
#8774=ORIENTED_EDGE ( 'NONE', *, *, #2647, .F. ) ;
#8826=CARTESIAN_POINT ( 'NONE',  ( -37.99999999999999289, -14.00000000000000888, -2.000000000000000000 ) ) ;
#8852=EDGE_CURVE ( 'NONE', #353, #7478, #10240, .T. ) ;
#8878=SURFACE_STYLE_FILL_AREA ( #10477 ) ;
#8889=EDGE_CURVE ( 'NONE', #9315, #6452, #2916, .T. ) ;
#8908=EDGE_LOOP ( 'NONE', ( #7964, #5177, #10024, #7297, #5201, #4729, #5761, #9692 ) ) ;
#8917=DIRECTION ( 'NONE',  ( 1.000000000000000000, 0.000000000000000000, 0.000000000000000000 ) ) ;
#8939=DIRECTION ( 'NONE',  ( -0.000000000000000000, 0.000000000000000000, 1.000000000000000000 ) ) ;
#8946=CIRCLE ( 'NONE', #242, 3.000000000000002665 ) ;
#8973=PRODUCT_CONTEXT ( 'NONE', #1001, 'mechanical' ) ;
#8986=( LENGTH_UNIT ( ) NAMED_UNIT ( * ) SI_UNIT ( .MILLI., .METRE. ) );
#8998=CARTESIAN_POINT ( 'NONE',  ( -57.99999999999998579, -10.00000000000000888, 0.000000000000000000 ) ) ;
#9002=DIRECTION ( 'NONE',  ( 0.7071067811865439090, 8.659560562354888485E-17, -0.7071067811865512365 ) ) ;
#9005=CARTESIAN_POINT ( 'NONE',  ( -44.00000000000000711, -14.00000000000000888, 0.000000000000000000 ) ) ;
#9021=AXIS2_PLACEMENT_3D ( 'NONE', #3439, #4994, #2673 ) ;
#9044=VECTOR ( 'NONE', #4169, 1000.000000000000000 ) ;
#9067=ORIENTED_EDGE ( 'NONE', *, *, #8852, .T. ) ;
#9089=ORIENTED_EDGE ( 'NONE', *, *, #508, .T. ) ;
#9097=VECTOR ( 'NONE', #4617, 1000.000000000000000 ) ;
#9106=VERTEX_POINT ( 'NONE', #3078 ) ;
#9109=DIRECTION ( 'NONE',  ( 1.000000000000000000, 0.000000000000000000, 0.000000000000000000 ) ) ;
#9118=CARTESIAN_POINT ( 'NONE',  ( -57.99999999999998579, -10.00000000000000888, 3.000000000000000000 ) ) ;
#9154=ADVANCED_FACE ( 'NONE', ( #8398 ), #9439, .F. ) ;
#9159=ORIENTED_EDGE ( 'NONE', *, *, #8113, .F. ) ;
#9205=VECTOR ( 'NONE', #5666, 1000.000000000000000 ) ;
#9210=DIRECTION ( 'NONE',  ( 0.000000000000000000, -0.000000000000000000, 1.000000000000000000 ) ) ;
#9221=VECTOR ( 'NONE', #6268, 1000.000000000000000 ) ;
#9227=AXIS2_PLACEMENT_3D ( 'NONE', #9731, #4444, #7905 ) ;
#9231=FACE_OUTER_BOUND ( 'NONE', #49, .T. ) ;
#9271=SHAPE_REPRESENTATION ( 'fine adjustment wheel', ( #2307 ), #5679 ) ;
#9274=EDGE_CURVE ( 'NONE', #2941, #6452, #7175, .T. ) ;
#9276=ORIENTED_EDGE ( 'NONE', *, *, #4087, .T. ) ;
#9299=ORIENTED_EDGE ( 'NONE', *, *, #153, .T. ) ;
#9315=VERTEX_POINT ( 'NONE', #1111 ) ;
#9345=PLANE ( 'NONE',  #4980 ) ;
#9355=VERTEX_POINT ( 'NONE', #7837 ) ;
#9362=EDGE_LOOP ( 'NONE', ( #300, #9695, #8484, #5884 ) ) ;
#9378=CYLINDRICAL_SURFACE ( 'NONE', #3906, 6.000000000000005329 ) ;
#9413=ORIENTED_EDGE ( 'NONE', *, *, #3094, .T. ) ;
#9439=PLANE ( 'NONE',  #9021 ) ;
#9502=DIRECTION ( 'NONE',  ( -0.000000000000000000, -0.000000000000000000, -1.000000000000000000 ) ) ;
#9544=ORIENTED_EDGE ( 'NONE', *, *, #8187, .F. ) ;
#9554=DIRECTION ( 'NONE',  ( -0.000000000000000000, -0.000000000000000000, -1.000000000000000000 ) ) ;
#9567=LINE ( 'NONE', #4505, #4127 ) ;
#9593=LINE ( 'NONE', #2819, #9221 ) ;
#9603=EDGE_LOOP ( 'NONE', ( #7470, #2712, #2691, #5545 ) ) ;
#9686=DIRECTION ( 'NONE',  ( 1.000000000000000000, 0.000000000000000000, 0.000000000000000000 ) ) ;
#9692=ORIENTED_EDGE ( 'NONE', *, *, #508, .F. ) ;
#9695=ORIENTED_EDGE ( 'NONE', *, *, #8073, .F. ) ;
#9702=FACE_OUTER_BOUND ( 'NONE', #10768, .T. ) ;
#9731=CARTESIAN_POINT ( 'NONE',  ( -37.99999999999999289, -14.00000000000000888, 0.000000000000000000 ) ) ;
#9782=ORIENTED_EDGE ( 'NONE', *, *, #4892, .T. ) ;
#9785=CARTESIAN_POINT ( 'NONE',  ( -42.47213595499957961, -10.00000000000000888, 3.000000000000000000 ) ) ;
#9794=CARTESIAN_POINT ( 'NONE',  ( -37.99999999999999289, -14.00000000000000888, 0.000000000000000000 ) ) ;
#9816=ADVANCED_FACE ( 'NONE', ( #1881 ), #7108, .F. ) ;
#9887=LINE ( 'NONE', #1391, #224 ) ;
#9899=AXIS2_PLACEMENT_3D ( 'NONE', #8108, #3878, #7269 ) ;
#9901=ORIENTED_EDGE ( 'NONE', *, *, #3305, .T. ) ;
#9914=LINE ( 'NONE', #10848, #2343 ) ;
#10024=ORIENTED_EDGE ( 'NONE', *, *, #2995, .T. ) ;
#10038=DIRECTION ( 'NONE',  ( 0.000000000000000000, -1.000000000000000000, 0.000000000000000000 ) ) ;
#10043=CARTESIAN_POINT ( 'NONE',  ( -44.00000000000000711, -14.00000000000000888, 3.000000000000000000 ) ) ;
#10060=CIRCLE ( 'NONE', #7585, 6.000000000000005329 ) ;
#10065=LINE ( 'NONE', #5846, #5178 ) ;
#10080=AXIS2_PLACEMENT_3D ( 'NONE', #5577, #2301, #531 ) ;
#10132=CARTESIAN_POINT ( 'NONE',  ( -49.99999999999998579, -10.00000000000000888, 3.000000000000000000 ) ) ;
#10158=DIRECTION ( 'NONE',  ( 0.000000000000000000, 0.000000000000000000, 1.000000000000000000 ) ) ;
#10223=ORIENTED_EDGE ( 'NONE', *, *, #6128, .T. ) ;
#10240=CIRCLE ( 'NONE', #5987, 6.000000000000005329 ) ;
#10255=CARTESIAN_POINT ( 'NONE',  ( -49.99999999999998579, -18.00000000000001066, 3.000000000000000000 ) ) ;
#10324=EDGE_CURVE ( 'NONE', #353, #9106, #1146, .T. ) ;
#10381=CARTESIAN_POINT ( 'NONE',  ( -37.99999999999999289, -14.00000000000000888, 5.000000000000000000 ) ) ;
#10419=FACE_OUTER_BOUND ( 'NONE', #6815, .T. ) ;
#10477=FILL_AREA_STYLE ('',( #4749 ) ) ;
#10514=DIRECTION ( 'NONE',  ( -0.000000000000000000, -0.000000000000000000, -1.000000000000000000 ) ) ;
#10615=CARTESIAN_POINT ( 'NONE',  ( -44.00000000000000000, -14.00000000000000888, 5.000000000000000000 ) ) ;
#10646=( NAMED_UNIT ( * ) PLANE_ANGLE_UNIT ( ) SI_UNIT ( $, .RADIAN. ) );
#10668=CARTESIAN_POINT ( 'NONE',  ( -32.99999999999997158, -14.00000000000000888, 5.000000000000000000 ) ) ;
#10706=( LENGTH_UNIT ( ) NAMED_UNIT ( * ) SI_UNIT ( .MILLI., .METRE. ) );
#10768=EDGE_LOOP ( 'NONE', ( #7506, #9299, #3069, #7543 ) ) ;
#10781=DIRECTION ( 'NONE',  ( 1.000000000000000000, 0.000000000000000000, 0.000000000000000000 ) ) ;
#10832=FACE_OUTER_BOUND ( 'NONE', #4488, .T. ) ;
#10848=CARTESIAN_POINT ( 'NONE',  ( -46.99999999999998579, -18.00000000000001066, 3.000000000000000000 ) ) ;
#10875=CARTESIAN_POINT ( 'NONE',  ( -49.99999999999998579, -10.00000000000000888, 3.000000000000000000 ) ) ;
#10889=CARTESIAN_POINT ( 'NONE',  ( -37.99999999999999289, -14.00000000000000888, 5.000000000000000000 ) ) ;
#10933=DIRECTION ( 'NONE',  ( -1.000000000000000000, 0.000000000000000000, 0.000000000000000000 ) ) ;
#11000=COLOUR_RGB('Light Blue',0.38,0.62,0.78);
#11001=FILL_AREA_STYLE_COLOUR('',#11000);
#11002=FILL_AREA_STYLE('',(#11001));
#11003=SURFACE_STYLE_FILL_AREA(#11002);
#11004=SURFACE_SIDE_STYLE('',(#11003));
#11005=SURFACE_STYLE_USAGE(.BOTH.,#11004);
#11006=PRESENTATION_STYLE_ASSIGNMENT((#11005));
ENDSEC;
END-ISO-10303-21;
